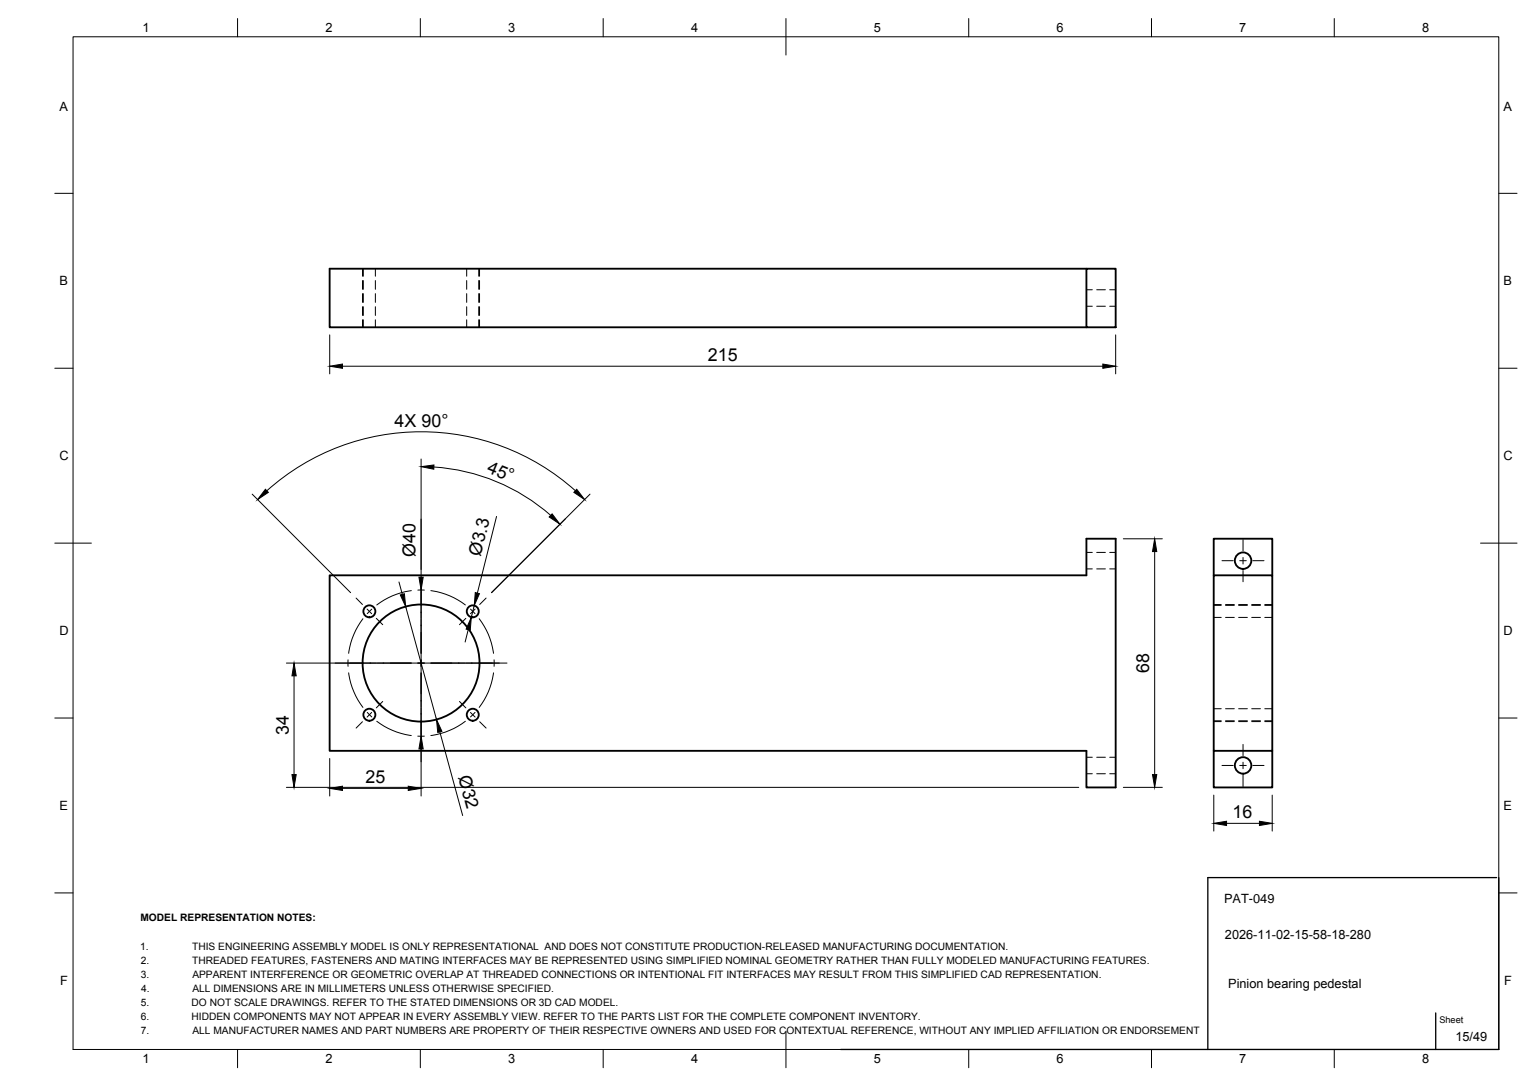
ISO-10303-21;
HEADER;
/* Generated by software containing ST-Developer
 * from STEP Tools, Inc. (www.steptools.com) 
 */

FILE_DESCRIPTION(
/* description */ ('Hand drill press frame (manual)'),
/* implementation_level */ '2;1');

FILE_NAME(
/* name */ 'Pinion bearing pedestal.step',
/* time_stamp */ '2026-10-28T03:25:28-07:00',
/* author */ (''),
/* organization */ (''),
/* preprocessor_version */ 'ST-DEVELOPER v20.2',
/* originating_system */ 'Autodesk Translation Framework v15.17.0.0',
/* authorisation */ '');

FILE_SCHEMA (('AUTOMOTIVE_DESIGN { 1 0 10303 214 3 1 1 }'));
ENDSEC;

DATA;
#10=MECHANICAL_DESIGN_GEOMETRIC_PRESENTATION_REPRESENTATION('',(#629),#33299);
#539=SHAPE_REPRESENTATION_RELATIONSHIP('SRR','None',#33498,#584);
#584=ADVANCED_BREP_SHAPE_REPRESENTATION('',(#681),#33260);
#629=STYLED_ITEM('',(#33814),#681);
#681=MANIFOLD_SOLID_BREP('Body1',#12647);
#764=FACE_BOUND('',#2219,.T.);
#765=FACE_BOUND('',#2221,.T.);
#766=FACE_BOUND('',#2225,.T.);
#767=FACE_BOUND('',#2226,.T.);
#768=FACE_BOUND('',#2227,.T.);
#769=FACE_BOUND('',#2228,.T.);
#770=FACE_BOUND('',#2229,.T.);
#771=FACE_BOUND('',#2232,.T.);
#772=FACE_BOUND('',#2233,.T.);
#773=FACE_BOUND('',#2234,.T.);
#774=FACE_BOUND('',#2235,.T.);
#775=FACE_BOUND('',#2236,.T.);
#776=FACE_BOUND('',#2240,.T.);
#777=FACE_BOUND('',#2241,.T.);
#983=PLANE('',#13453);
#984=PLANE('',#13454);
#985=PLANE('',#13455);
#986=PLANE('',#13456);
#987=PLANE('',#13457);
#988=PLANE('',#13458);
#989=PLANE('',#13459);
#990=PLANE('',#13460);
#991=PLANE('',#13461);
#992=PLANE('',#13462);
#1478=FACE_OUTER_BOUND('',#2211,.T.);
#1479=FACE_OUTER_BOUND('',#2212,.T.);
#1480=FACE_OUTER_BOUND('',#2213,.T.);
#1481=FACE_OUTER_BOUND('',#2214,.T.);
#1482=FACE_OUTER_BOUND('',#2215,.T.);
#1483=FACE_OUTER_BOUND('',#2216,.T.);
#1484=FACE_OUTER_BOUND('',#2217,.T.);
#1485=FACE_OUTER_BOUND('',#2218,.T.);
#1486=FACE_OUTER_BOUND('',#2220,.T.);
#1487=FACE_OUTER_BOUND('',#2222,.T.);
#1488=FACE_OUTER_BOUND('',#2223,.T.);
#1489=FACE_OUTER_BOUND('',#2224,.T.);
#1490=FACE_OUTER_BOUND('',#2230,.T.);
#1491=FACE_OUTER_BOUND('',#2231,.T.);
#1492=FACE_OUTER_BOUND('',#2237,.T.);
#1493=FACE_OUTER_BOUND('',#2238,.T.);
#1494=FACE_OUTER_BOUND('',#2239,.T.);
#2211=EDGE_LOOP('',(#9089,#9090,#9091,#9092));
#2212=EDGE_LOOP('',(#9093,#9094,#9095,#9096));
#2213=EDGE_LOOP('',(#9097,#9098,#9099,#9100));
#2214=EDGE_LOOP('',(#9101,#9102,#9103,#9104));
#2215=EDGE_LOOP('',(#9105,#9106,#9107,#9108));
#2216=EDGE_LOOP('',(#9109,#9110,#9111,#9112));
#2217=EDGE_LOOP('',(#9113,#9114,#9115,#9116));
#2218=EDGE_LOOP('',(#9117,#9118,#9119,#9120));
#2219=EDGE_LOOP('',(#9121));
#2220=EDGE_LOOP('',(#9122,#9123,#9124,#9125));
#2221=EDGE_LOOP('',(#9126));
#2222=EDGE_LOOP('',(#9127,#9128,#9129,#9130));
#2223=EDGE_LOOP('',(#9131,#9132,#9133,#9134));
#2224=EDGE_LOOP('',(#9135,#9136,#9137,#9138,#9139,#9140,#9141,#9142));
#2225=EDGE_LOOP('',(#9143));
#2226=EDGE_LOOP('',(#9144));
#2227=EDGE_LOOP('',(#9145));
#2228=EDGE_LOOP('',(#9146));
#2229=EDGE_LOOP('',(#9147));
#2230=EDGE_LOOP('',(#9148,#9149,#9150,#9151));
#2231=EDGE_LOOP('',(#9152,#9153,#9154,#9155,#9156,#9157,#9158,#9159));
#2232=EDGE_LOOP('',(#9160));
#2233=EDGE_LOOP('',(#9161));
#2234=EDGE_LOOP('',(#9162));
#2235=EDGE_LOOP('',(#9163));
#2236=EDGE_LOOP('',(#9164));
#2237=EDGE_LOOP('',(#9165,#9166,#9167,#9168));
#2238=EDGE_LOOP('',(#9169,#9170,#9171,#9172));
#2239=EDGE_LOOP('',(#9173,#9174,#9175,#9176));
#2240=EDGE_LOOP('',(#9177));
#2241=EDGE_LOOP('',(#9178));
#3111=LINE('',#18786,#4276);
#3112=LINE('',#18792,#4277);
#3113=LINE('',#18798,#4278);
#3114=LINE('',#18804,#4279);
#3115=LINE('',#18810,#4280);
#3116=LINE('',#18816,#4281);
#3117=LINE('',#18822,#4282);
#3118=LINE('',#18827,#4283);
#3119=LINE('',#18829,#4284);
#3120=LINE('',#18831,#4285);
#3121=LINE('',#18832,#4286);
#3122=LINE('',#18836,#4287);
#3123=LINE('',#18838,#4288);
#3124=LINE('',#18840,#4289);
#3125=LINE('',#18841,#4290);
#3126=LINE('',#18844,#4291);
#3127=LINE('',#18846,#4292);
#3128=LINE('',#18847,#4293);
#3129=LINE('',#18850,#4294);
#3130=LINE('',#18852,#4295);
#3131=LINE('',#18853,#4296);
#3132=LINE('',#18856,#4297);
#3133=LINE('',#18858,#4298);
#3134=LINE('',#18859,#4299);
#3135=LINE('',#18860,#4300);
#3136=LINE('',#18863,#4301);
#3137=LINE('',#18864,#4302);
#3138=LINE('',#18867,#4303);
#3139=LINE('',#18868,#4304);
#3140=LINE('',#18869,#4305);
#3141=LINE('',#18871,#4306);
#4276=VECTOR('',#15086,0.165);
#4277=VECTOR('',#15093,0.165);
#4278=VECTOR('',#15100,0.165);
#4279=VECTOR('',#15107,0.165);
#4280=VECTOR('',#15114,0.225);
#4281=VECTOR('',#15121,0.225);
#4282=VECTOR('',#15128,1.6);
#4283=VECTOR('',#15133,1.);
#4284=VECTOR('',#15134,1.);
#4285=VECTOR('',#15135,1.);
#4286=VECTOR('',#15136,1.);
#4287=VECTOR('',#15139,1.);
#4288=VECTOR('',#15140,1.);
#4289=VECTOR('',#15141,1.);
#4290=VECTOR('',#15142,1.);
#4291=VECTOR('',#15145,1.);
#4292=VECTOR('',#15146,1.);
#4293=VECTOR('',#15147,1.);
#4294=VECTOR('',#15150,1.);
#4295=VECTOR('',#15151,1.);
#4296=VECTOR('',#15152,1.);
#4297=VECTOR('',#15155,1.);
#4298=VECTOR('',#15156,1.);
#4299=VECTOR('',#15157,1.);
#4300=VECTOR('',#15158,1.);
#4301=VECTOR('',#15161,1.);
#4302=VECTOR('',#15162,1.);
#4303=VECTOR('',#15165,1.);
#4304=VECTOR('',#15166,1.);
#4305=VECTOR('',#15167,1.);
#4306=VECTOR('',#15170,1.);
#5306=CIRCLE('',#13433,0.165);
#5307=CIRCLE('',#13434,0.165);
#5308=CIRCLE('',#13436,0.165);
#5309=CIRCLE('',#13437,0.165);
#5310=CIRCLE('',#13439,0.165);
#5311=CIRCLE('',#13440,0.165);
#5312=CIRCLE('',#13442,0.165);
#5313=CIRCLE('',#13443,0.165);
#5314=CIRCLE('',#13445,0.225);
#5315=CIRCLE('',#13446,0.225);
#5316=CIRCLE('',#13448,0.225);
#5317=CIRCLE('',#13449,0.225);
#5318=CIRCLE('',#13451,1.6);
#5319=CIRCLE('',#13452,1.6);
#5836=VERTEX_POINT('',#18783);
#5837=VERTEX_POINT('',#18785);
#5838=VERTEX_POINT('',#18789);
#5839=VERTEX_POINT('',#18791);
#5840=VERTEX_POINT('',#18795);
#5841=VERTEX_POINT('',#18797);
#5842=VERTEX_POINT('',#18801);
#5843=VERTEX_POINT('',#18803);
#5844=VERTEX_POINT('',#18807);
#5845=VERTEX_POINT('',#18809);
#5846=VERTEX_POINT('',#18813);
#5847=VERTEX_POINT('',#18815);
#5848=VERTEX_POINT('',#18819);
#5849=VERTEX_POINT('',#18821);
#5850=VERTEX_POINT('',#18825);
#5851=VERTEX_POINT('',#18826);
#5852=VERTEX_POINT('',#18828);
#5853=VERTEX_POINT('',#18830);
#5854=VERTEX_POINT('',#18834);
#5855=VERTEX_POINT('',#18835);
#5856=VERTEX_POINT('',#18837);
#5857=VERTEX_POINT('',#18839);
#5858=VERTEX_POINT('',#18843);
#5859=VERTEX_POINT('',#18845);
#5860=VERTEX_POINT('',#18849);
#5861=VERTEX_POINT('',#18851);
#5862=VERTEX_POINT('',#18855);
#5863=VERTEX_POINT('',#18857);
#5864=VERTEX_POINT('',#18862);
#5865=VERTEX_POINT('',#18866);
#7073=EDGE_CURVE('',#5836,#5836,#5306,.T.);
#7074=EDGE_CURVE('',#5836,#5837,#3111,.T.);
#7075=EDGE_CURVE('',#5837,#5837,#5307,.T.);
#7076=EDGE_CURVE('',#5838,#5838,#5308,.T.);
#7077=EDGE_CURVE('',#5838,#5839,#3112,.T.);
#7078=EDGE_CURVE('',#5839,#5839,#5309,.T.);
#7079=EDGE_CURVE('',#5840,#5840,#5310,.T.);
#7080=EDGE_CURVE('',#5840,#5841,#3113,.T.);
#7081=EDGE_CURVE('',#5841,#5841,#5311,.T.);
#7082=EDGE_CURVE('',#5842,#5842,#5312,.T.);
#7083=EDGE_CURVE('',#5842,#5843,#3114,.T.);
#7084=EDGE_CURVE('',#5843,#5843,#5313,.T.);
#7085=EDGE_CURVE('',#5844,#5844,#5314,.T.);
#7086=EDGE_CURVE('',#5844,#5845,#3115,.T.);
#7087=EDGE_CURVE('',#5845,#5845,#5315,.T.);
#7088=EDGE_CURVE('',#5846,#5846,#5316,.T.);
#7089=EDGE_CURVE('',#5846,#5847,#3116,.T.);
#7090=EDGE_CURVE('',#5847,#5847,#5317,.T.);
#7091=EDGE_CURVE('',#5848,#5848,#5318,.T.);
#7092=EDGE_CURVE('',#5848,#5849,#3117,.T.);
#7093=EDGE_CURVE('',#5849,#5849,#5319,.T.);
#7094=EDGE_CURVE('',#5850,#5851,#3118,.T.);
#7095=EDGE_CURVE('',#5852,#5850,#3119,.T.);
#7096=EDGE_CURVE('',#5852,#5853,#3120,.T.);
#7097=EDGE_CURVE('',#5851,#5853,#3121,.T.);
#7098=EDGE_CURVE('',#5854,#5855,#3122,.T.);
#7099=EDGE_CURVE('',#5856,#5854,#3123,.T.);
#7100=EDGE_CURVE('',#5857,#5856,#3124,.T.);
#7101=EDGE_CURVE('',#5855,#5857,#3125,.T.);
#7102=EDGE_CURVE('',#5857,#5858,#3126,.T.);
#7103=EDGE_CURVE('',#5859,#5856,#3127,.T.);
#7104=EDGE_CURVE('',#5858,#5859,#3128,.T.);
#7105=EDGE_CURVE('',#5860,#5852,#3129,.T.);
#7106=EDGE_CURVE('',#5860,#5861,#3130,.T.);
#7107=EDGE_CURVE('',#5853,#5861,#3131,.T.);
#7108=EDGE_CURVE('',#5850,#5862,#3132,.T.);
#7109=EDGE_CURVE('',#5863,#5862,#3133,.T.);
#7110=EDGE_CURVE('',#5855,#5863,#3134,.T.);
#7111=EDGE_CURVE('',#5858,#5860,#3135,.T.);
#7112=EDGE_CURVE('',#5851,#5864,#3136,.T.);
#7113=EDGE_CURVE('',#5862,#5864,#3137,.T.);
#7114=EDGE_CURVE('',#5854,#5865,#3138,.T.);
#7115=EDGE_CURVE('',#5864,#5865,#3139,.T.);
#7116=EDGE_CURVE('',#5861,#5859,#3140,.T.);
#7117=EDGE_CURVE('',#5865,#5863,#3141,.T.);
#9089=ORIENTED_EDGE('',*,*,#7073,.F.);
#9090=ORIENTED_EDGE('',*,*,#7074,.T.);
#9091=ORIENTED_EDGE('',*,*,#7075,.F.);
#9092=ORIENTED_EDGE('',*,*,#7074,.F.);
#9093=ORIENTED_EDGE('',*,*,#7076,.F.);
#9094=ORIENTED_EDGE('',*,*,#7077,.T.);
#9095=ORIENTED_EDGE('',*,*,#7078,.F.);
#9096=ORIENTED_EDGE('',*,*,#7077,.F.);
#9097=ORIENTED_EDGE('',*,*,#7079,.F.);
#9098=ORIENTED_EDGE('',*,*,#7080,.T.);
#9099=ORIENTED_EDGE('',*,*,#7081,.F.);
#9100=ORIENTED_EDGE('',*,*,#7080,.F.);
#9101=ORIENTED_EDGE('',*,*,#7082,.F.);
#9102=ORIENTED_EDGE('',*,*,#7083,.T.);
#9103=ORIENTED_EDGE('',*,*,#7084,.F.);
#9104=ORIENTED_EDGE('',*,*,#7083,.F.);
#9105=ORIENTED_EDGE('',*,*,#7085,.F.);
#9106=ORIENTED_EDGE('',*,*,#7086,.T.);
#9107=ORIENTED_EDGE('',*,*,#7087,.F.);
#9108=ORIENTED_EDGE('',*,*,#7086,.F.);
#9109=ORIENTED_EDGE('',*,*,#7088,.F.);
#9110=ORIENTED_EDGE('',*,*,#7089,.T.);
#9111=ORIENTED_EDGE('',*,*,#7090,.F.);
#9112=ORIENTED_EDGE('',*,*,#7089,.F.);
#9113=ORIENTED_EDGE('',*,*,#7091,.F.);
#9114=ORIENTED_EDGE('',*,*,#7092,.T.);
#9115=ORIENTED_EDGE('',*,*,#7093,.F.);
#9116=ORIENTED_EDGE('',*,*,#7092,.F.);
#9117=ORIENTED_EDGE('',*,*,#7094,.F.);
#9118=ORIENTED_EDGE('',*,*,#7095,.F.);
#9119=ORIENTED_EDGE('',*,*,#7096,.T.);
#9120=ORIENTED_EDGE('',*,*,#7097,.F.);
#9121=ORIENTED_EDGE('',*,*,#7090,.T.);
#9122=ORIENTED_EDGE('',*,*,#7098,.F.);
#9123=ORIENTED_EDGE('',*,*,#7099,.F.);
#9124=ORIENTED_EDGE('',*,*,#7100,.F.);
#9125=ORIENTED_EDGE('',*,*,#7101,.F.);
#9126=ORIENTED_EDGE('',*,*,#7087,.T.);
#9127=ORIENTED_EDGE('',*,*,#7102,.F.);
#9128=ORIENTED_EDGE('',*,*,#7100,.T.);
#9129=ORIENTED_EDGE('',*,*,#7103,.F.);
#9130=ORIENTED_EDGE('',*,*,#7104,.F.);
#9131=ORIENTED_EDGE('',*,*,#7105,.F.);
#9132=ORIENTED_EDGE('',*,*,#7106,.T.);
#9133=ORIENTED_EDGE('',*,*,#7107,.F.);
#9134=ORIENTED_EDGE('',*,*,#7096,.F.);
#9135=ORIENTED_EDGE('',*,*,#7108,.T.);
#9136=ORIENTED_EDGE('',*,*,#7109,.F.);
#9137=ORIENTED_EDGE('',*,*,#7110,.F.);
#9138=ORIENTED_EDGE('',*,*,#7101,.T.);
#9139=ORIENTED_EDGE('',*,*,#7102,.T.);
#9140=ORIENTED_EDGE('',*,*,#7111,.T.);
#9141=ORIENTED_EDGE('',*,*,#7105,.T.);
#9142=ORIENTED_EDGE('',*,*,#7095,.T.);
#9143=ORIENTED_EDGE('',*,*,#7091,.T.);
#9144=ORIENTED_EDGE('',*,*,#7082,.T.);
#9145=ORIENTED_EDGE('',*,*,#7079,.T.);
#9146=ORIENTED_EDGE('',*,*,#7076,.T.);
#9147=ORIENTED_EDGE('',*,*,#7073,.T.);
#9148=ORIENTED_EDGE('',*,*,#7094,.T.);
#9149=ORIENTED_EDGE('',*,*,#7112,.T.);
#9150=ORIENTED_EDGE('',*,*,#7113,.F.);
#9151=ORIENTED_EDGE('',*,*,#7108,.F.);
#9152=ORIENTED_EDGE('',*,*,#7114,.T.);
#9153=ORIENTED_EDGE('',*,*,#7115,.F.);
#9154=ORIENTED_EDGE('',*,*,#7112,.F.);
#9155=ORIENTED_EDGE('',*,*,#7097,.T.);
#9156=ORIENTED_EDGE('',*,*,#7107,.T.);
#9157=ORIENTED_EDGE('',*,*,#7116,.T.);
#9158=ORIENTED_EDGE('',*,*,#7103,.T.);
#9159=ORIENTED_EDGE('',*,*,#7099,.T.);
#9160=ORIENTED_EDGE('',*,*,#7093,.T.);
#9161=ORIENTED_EDGE('',*,*,#7084,.T.);
#9162=ORIENTED_EDGE('',*,*,#7081,.T.);
#9163=ORIENTED_EDGE('',*,*,#7078,.T.);
#9164=ORIENTED_EDGE('',*,*,#7075,.T.);
#9165=ORIENTED_EDGE('',*,*,#7098,.T.);
#9166=ORIENTED_EDGE('',*,*,#7110,.T.);
#9167=ORIENTED_EDGE('',*,*,#7117,.F.);
#9168=ORIENTED_EDGE('',*,*,#7114,.F.);
#9169=ORIENTED_EDGE('',*,*,#7117,.T.);
#9170=ORIENTED_EDGE('',*,*,#7109,.T.);
#9171=ORIENTED_EDGE('',*,*,#7113,.T.);
#9172=ORIENTED_EDGE('',*,*,#7115,.T.);
#9173=ORIENTED_EDGE('',*,*,#7116,.F.);
#9174=ORIENTED_EDGE('',*,*,#7106,.F.);
#9175=ORIENTED_EDGE('',*,*,#7111,.F.);
#9176=ORIENTED_EDGE('',*,*,#7104,.T.);
#9177=ORIENTED_EDGE('',*,*,#7085,.T.);
#9178=ORIENTED_EDGE('',*,*,#7088,.T.);
#11828=CYLINDRICAL_SURFACE('',#13432,0.165);
#11829=CYLINDRICAL_SURFACE('',#13435,0.165);
#11830=CYLINDRICAL_SURFACE('',#13438,0.165);
#11831=CYLINDRICAL_SURFACE('',#13441,0.165);
#11832=CYLINDRICAL_SURFACE('',#13444,0.225);
#11833=CYLINDRICAL_SURFACE('',#13447,0.225);
#11834=CYLINDRICAL_SURFACE('',#13450,1.6);
#12087=ADVANCED_FACE('',(#1478),#11828,.F.);
#12088=ADVANCED_FACE('',(#1479),#11829,.F.);
#12089=ADVANCED_FACE('',(#1480),#11830,.F.);
#12090=ADVANCED_FACE('',(#1481),#11831,.F.);
#12091=ADVANCED_FACE('',(#1482),#11832,.F.);
#12092=ADVANCED_FACE('',(#1483),#11833,.F.);
#12093=ADVANCED_FACE('',(#1484),#11834,.F.);
#12094=ADVANCED_FACE('',(#1485,#764),#983,.T.);
#12095=ADVANCED_FACE('',(#1486,#765),#984,.T.);
#12096=ADVANCED_FACE('',(#1487),#985,.T.);
#12097=ADVANCED_FACE('',(#1488),#986,.T.);
#12098=ADVANCED_FACE('',(#1489,#766,#767,#768,#769,#770),#987,.T.);
#12099=ADVANCED_FACE('',(#1490),#988,.T.);
#12100=ADVANCED_FACE('',(#1491,#771,#772,#773,#774,#775),#989,.T.);
#12101=ADVANCED_FACE('',(#1492),#990,.T.);
#12102=ADVANCED_FACE('',(#1493),#991,.T.);
#12103=ADVANCED_FACE('',(#1494,#776,#777),#992,.F.);
#12647=CLOSED_SHELL('',(#12087,#12088,#12089,#12090,#12091,#12092,#12093,
#12094,#12095,#12096,#12097,#12098,#12099,#12100,#12101,#12102,#12103));
#13431=AXIS2_PLACEMENT_3D('',#18781,#15080,#15081);
#13432=AXIS2_PLACEMENT_3D('',#18782,#15082,#15083);
#13433=AXIS2_PLACEMENT_3D('',#18784,#15084,#15085);
#13434=AXIS2_PLACEMENT_3D('',#18787,#15087,#15088);
#13435=AXIS2_PLACEMENT_3D('',#18788,#15089,#15090);
#13436=AXIS2_PLACEMENT_3D('',#18790,#15091,#15092);
#13437=AXIS2_PLACEMENT_3D('',#18793,#15094,#15095);
#13438=AXIS2_PLACEMENT_3D('',#18794,#15096,#15097);
#13439=AXIS2_PLACEMENT_3D('',#18796,#15098,#15099);
#13440=AXIS2_PLACEMENT_3D('',#18799,#15101,#15102);
#13441=AXIS2_PLACEMENT_3D('',#18800,#15103,#15104);
#13442=AXIS2_PLACEMENT_3D('',#18802,#15105,#15106);
#13443=AXIS2_PLACEMENT_3D('',#18805,#15108,#15109);
#13444=AXIS2_PLACEMENT_3D('',#18806,#15110,#15111);
#13445=AXIS2_PLACEMENT_3D('',#18808,#15112,#15113);
#13446=AXIS2_PLACEMENT_3D('',#18811,#15115,#15116);
#13447=AXIS2_PLACEMENT_3D('',#18812,#15117,#15118);
#13448=AXIS2_PLACEMENT_3D('',#18814,#15119,#15120);
#13449=AXIS2_PLACEMENT_3D('',#18817,#15122,#15123);
#13450=AXIS2_PLACEMENT_3D('',#18818,#15124,#15125);
#13451=AXIS2_PLACEMENT_3D('',#18820,#15126,#15127);
#13452=AXIS2_PLACEMENT_3D('',#18823,#15129,#15130);
#13453=AXIS2_PLACEMENT_3D('',#18824,#15131,#15132);
#13454=AXIS2_PLACEMENT_3D('',#18833,#15137,#15138);
#13455=AXIS2_PLACEMENT_3D('',#18842,#15143,#15144);
#13456=AXIS2_PLACEMENT_3D('',#18848,#15148,#15149);
#13457=AXIS2_PLACEMENT_3D('',#18854,#15153,#15154);
#13458=AXIS2_PLACEMENT_3D('',#18861,#15159,#15160);
#13459=AXIS2_PLACEMENT_3D('',#18865,#15163,#15164);
#13460=AXIS2_PLACEMENT_3D('',#18870,#15168,#15169);
#13461=AXIS2_PLACEMENT_3D('',#18872,#15171,#15172);
#13462=AXIS2_PLACEMENT_3D('',#18873,#15173,#15174);
#15080=DIRECTION('axis',(0.,0.,1.));
#15081=DIRECTION('refdir',(1.,0.,0.));
#15082=DIRECTION('center_axis',(0.,1.,0.));
#15083=DIRECTION('ref_axis',(1.,0.,0.));
#15084=DIRECTION('center_axis',(0.,1.,0.));
#15085=DIRECTION('ref_axis',(1.,0.,0.));
#15086=DIRECTION('',(0.,1.,0.));
#15087=DIRECTION('center_axis',(0.,-1.,0.));
#15088=DIRECTION('ref_axis',(1.,0.,0.));
#15089=DIRECTION('center_axis',(0.,1.,0.));
#15090=DIRECTION('ref_axis',(1.,0.,0.));
#15091=DIRECTION('center_axis',(0.,1.,0.));
#15092=DIRECTION('ref_axis',(1.,0.,0.));
#15093=DIRECTION('',(0.,1.,0.));
#15094=DIRECTION('center_axis',(0.,-1.,0.));
#15095=DIRECTION('ref_axis',(1.,0.,0.));
#15096=DIRECTION('center_axis',(0.,1.,0.));
#15097=DIRECTION('ref_axis',(1.,0.,0.));
#15098=DIRECTION('center_axis',(0.,1.,0.));
#15099=DIRECTION('ref_axis',(1.,0.,0.));
#15100=DIRECTION('',(0.,1.,0.));
#15101=DIRECTION('center_axis',(0.,-1.,0.));
#15102=DIRECTION('ref_axis',(1.,0.,0.));
#15103=DIRECTION('center_axis',(0.,1.,0.));
#15104=DIRECTION('ref_axis',(1.,0.,0.));
#15105=DIRECTION('center_axis',(0.,1.,0.));
#15106=DIRECTION('ref_axis',(1.,0.,0.));
#15107=DIRECTION('',(0.,1.,0.));
#15108=DIRECTION('center_axis',(0.,-1.,0.));
#15109=DIRECTION('ref_axis',(1.,0.,0.));
#15110=DIRECTION('center_axis',(0.,0.,1.));
#15111=DIRECTION('ref_axis',(1.,0.,0.));
#15112=DIRECTION('center_axis',(0.,0.,1.));
#15113=DIRECTION('ref_axis',(1.,0.,0.));
#15114=DIRECTION('',(0.,0.,1.));
#15115=DIRECTION('center_axis',(0.,0.,-1.));
#15116=DIRECTION('ref_axis',(1.,0.,0.));
#15117=DIRECTION('center_axis',(0.,0.,1.));
#15118=DIRECTION('ref_axis',(1.,0.,0.));
#15119=DIRECTION('center_axis',(0.,0.,1.));
#15120=DIRECTION('ref_axis',(1.,0.,0.));
#15121=DIRECTION('',(0.,0.,1.));
#15122=DIRECTION('center_axis',(0.,0.,-1.));
#15123=DIRECTION('ref_axis',(1.,0.,0.));
#15124=DIRECTION('center_axis',(0.,1.,0.));
#15125=DIRECTION('ref_axis',(1.,0.,0.));
#15126=DIRECTION('center_axis',(0.,1.,0.));
#15127=DIRECTION('ref_axis',(1.,0.,0.));
#15128=DIRECTION('',(0.,1.,0.));
#15129=DIRECTION('center_axis',(0.,-1.,0.));
#15130=DIRECTION('ref_axis',(1.,0.,0.));
#15131=DIRECTION('center_axis',(0.,0.,1.));
#15132=DIRECTION('ref_axis',(1.,0.,0.));
#15133=DIRECTION('',(0.,1.,0.));
#15134=DIRECTION('',(-1.,0.,0.));
#15135=DIRECTION('',(0.,1.,0.));
#15136=DIRECTION('',(1.,0.,0.));
#15137=DIRECTION('center_axis',(0.,0.,1.));
#15138=DIRECTION('ref_axis',(1.,0.,0.));
#15139=DIRECTION('',(0.,-1.,0.));
#15140=DIRECTION('',(1.,0.,0.));
#15141=DIRECTION('',(0.,1.,0.));
#15142=DIRECTION('',(-1.,0.,0.));
#15143=DIRECTION('center_axis',(-1.,0.,0.));
#15144=DIRECTION('ref_axis',(0.,0.,1.));
#15145=DIRECTION('',(0.,0.,-1.));
#15146=DIRECTION('',(0.,0.,1.));
#15147=DIRECTION('',(0.,1.,0.));
#15148=DIRECTION('center_axis',(1.,0.,0.));
#15149=DIRECTION('ref_axis',(0.,0.,-1.));
#15150=DIRECTION('',(0.,0.,1.));
#15151=DIRECTION('',(0.,1.,0.));
#15152=DIRECTION('',(0.,0.,-1.));
#15153=DIRECTION('center_axis',(0.,-1.,0.));
#15154=DIRECTION('ref_axis',(1.,0.,0.));
#15155=DIRECTION('',(0.,0.,1.));
#15156=DIRECTION('',(1.,0.,0.));
#15157=DIRECTION('',(0.,0.,1.));
#15158=DIRECTION('',(1.,0.,0.));
#15159=DIRECTION('center_axis',(1.,0.,0.));
#15160=DIRECTION('ref_axis',(0.,1.,0.));
#15161=DIRECTION('',(0.,0.,1.));
#15162=DIRECTION('',(0.,1.,0.));
#15163=DIRECTION('center_axis',(0.,1.,0.));
#15164=DIRECTION('ref_axis',(-1.,0.,0.));
#15165=DIRECTION('',(0.,0.,1.));
#15166=DIRECTION('',(-1.,0.,0.));
#15167=DIRECTION('',(-1.,0.,0.));
#15168=DIRECTION('center_axis',(-1.,0.,0.));
#15169=DIRECTION('ref_axis',(0.,-1.,0.));
#15170=DIRECTION('',(0.,-1.,0.));
#15171=DIRECTION('center_axis',(0.,0.,1.));
#15172=DIRECTION('ref_axis',(1.,0.,0.));
#15173=DIRECTION('center_axis',(0.,0.,1.));
#15174=DIRECTION('ref_axis',(1.,0.,0.));
#18781=CARTESIAN_POINT('',(0.,0.,0.));
#18782=CARTESIAN_POINT('Origin',(-4.66421356237309,-3.9,18.5857864376269));
#18783=CARTESIAN_POINT('',(-4.82921356237309,-3.8,18.5857864376269));
#18784=CARTESIAN_POINT('Origin',(-4.66421356237309,-3.8,18.5857864376269));
#18785=CARTESIAN_POINT('',(-4.82921356237309,-2.2,18.5857864376269));
#18786=CARTESIAN_POINT('',(-4.82921356237309,-3.9,18.5857864376269));
#18787=CARTESIAN_POINT('Origin',(-4.66421356237309,-2.2,18.5857864376269));
#18788=CARTESIAN_POINT('Origin',(-4.66421356237309,-3.9,21.4142135623731));
#18789=CARTESIAN_POINT('',(-4.82921356237309,-3.8,21.4142135623731));
#18790=CARTESIAN_POINT('Origin',(-4.66421356237309,-3.8,21.4142135623731));
#18791=CARTESIAN_POINT('',(-4.82921356237309,-2.2,21.4142135623731));
#18792=CARTESIAN_POINT('',(-4.82921356237309,-3.9,21.4142135623731));
#18793=CARTESIAN_POINT('Origin',(-4.66421356237309,-2.2,21.4142135623731));
#18794=CARTESIAN_POINT('Origin',(-1.8357864376269,-3.9,21.4142135623731));
#18795=CARTESIAN_POINT('',(-2.00078643762691,-3.8,21.4142135623731));
#18796=CARTESIAN_POINT('Origin',(-1.8357864376269,-3.8,21.4142135623731));
#18797=CARTESIAN_POINT('',(-2.00078643762691,-2.2,21.4142135623731));
#18798=CARTESIAN_POINT('',(-2.00078643762691,-3.9,21.4142135623731));
#18799=CARTESIAN_POINT('Origin',(-1.8357864376269,-2.2,21.4142135623731));
#18800=CARTESIAN_POINT('Origin',(-1.83578643762691,-3.9,18.5857864376269));
#18801=CARTESIAN_POINT('',(-2.00078643762691,-3.8,18.5857864376269));
#18802=CARTESIAN_POINT('Origin',(-1.83578643762691,-3.8,18.5857864376269));
#18803=CARTESIAN_POINT('',(-2.00078643762691,-2.2,18.5857864376269));
#18804=CARTESIAN_POINT('',(-2.00078643762691,-3.9,18.5857864376269));
#18805=CARTESIAN_POINT('Origin',(-1.83578643762691,-2.2,18.5857864376269));
#18806=CARTESIAN_POINT('Origin',(-6.05,-3.,0.9));
#18807=CARTESIAN_POINT('',(-6.275,-3.,1.));
#18808=CARTESIAN_POINT('Origin',(-6.05,-3.,1.));
#18809=CARTESIAN_POINT('',(-6.275,-3.,1.8));
#18810=CARTESIAN_POINT('',(-6.275,-3.,0.9));
#18811=CARTESIAN_POINT('Origin',(-6.05,-3.,1.8));
#18812=CARTESIAN_POINT('Origin',(-0.45,-3.,0.9));
#18813=CARTESIAN_POINT('',(-0.675,-3.,1.));
#18814=CARTESIAN_POINT('Origin',(-0.45,-3.,1.));
#18815=CARTESIAN_POINT('',(-0.675,-3.,1.8));
#18816=CARTESIAN_POINT('',(-0.675,-3.,0.9));
#18817=CARTESIAN_POINT('Origin',(-0.45,-3.,1.8));
#18818=CARTESIAN_POINT('Origin',(-3.25,-3.9,20.));
#18819=CARTESIAN_POINT('',(-4.85,-3.8,20.));
#18820=CARTESIAN_POINT('Origin',(-3.25,-3.8,20.));
#18821=CARTESIAN_POINT('',(-4.85,-2.2,20.));
#18822=CARTESIAN_POINT('',(-4.85,-3.9,20.));
#18823=CARTESIAN_POINT('Origin',(-3.25,-2.2,20.));
#18824=CARTESIAN_POINT('Origin',(-6.65,-3.8,1.8));
#18825=CARTESIAN_POINT('',(-0.85,-3.8,1.8));
#18826=CARTESIAN_POINT('',(-0.85,-2.2,1.8));
#18827=CARTESIAN_POINT('',(-0.85,-3.8,1.8));
#18828=CARTESIAN_POINT('',(0.15,-3.8,1.8));
#18829=CARTESIAN_POINT('',(0.15,-3.8,1.8));
#18830=CARTESIAN_POINT('',(0.15,-2.2,1.8));
#18831=CARTESIAN_POINT('',(0.15,-3.8,1.8));
#18832=CARTESIAN_POINT('',(0.15,-2.2,1.8));
#18833=CARTESIAN_POINT('Origin',(-6.65,-3.8,1.8));
#18834=CARTESIAN_POINT('',(-5.65,-2.2,1.8));
#18835=CARTESIAN_POINT('',(-5.65,-3.8,1.8));
#18836=CARTESIAN_POINT('',(-5.65,-3.,1.8));
#18837=CARTESIAN_POINT('',(-6.65,-2.2,1.8));
#18838=CARTESIAN_POINT('',(0.15,-2.2,1.8));
#18839=CARTESIAN_POINT('',(-6.65,-3.8,1.8));
#18840=CARTESIAN_POINT('',(-6.65,-3.8,1.8));
#18841=CARTESIAN_POINT('',(0.15,-3.8,1.8));
#18842=CARTESIAN_POINT('Origin',(-6.65,-3.8,1.));
#18843=CARTESIAN_POINT('',(-6.65,-3.8,1.));
#18844=CARTESIAN_POINT('',(-6.65,-3.8,1.8));
#18845=CARTESIAN_POINT('',(-6.65,-2.2,1.));
#18846=CARTESIAN_POINT('',(-6.65,-2.2,1.8));
#18847=CARTESIAN_POINT('',(-6.65,-3.8,1.));
#18848=CARTESIAN_POINT('Origin',(0.15,-3.8,1.8));
#18849=CARTESIAN_POINT('',(0.15,-3.8,1.));
#18850=CARTESIAN_POINT('',(0.15,-3.8,1.));
#18851=CARTESIAN_POINT('',(0.15,-2.2,1.));
#18852=CARTESIAN_POINT('',(0.15,-3.8,1.));
#18853=CARTESIAN_POINT('',(0.15,-2.2,1.));
#18854=CARTESIAN_POINT('Origin',(-5.65,-3.8,1.));
#18855=CARTESIAN_POINT('',(-0.85,-3.8,22.5));
#18856=CARTESIAN_POINT('',(-0.85,-3.8,1.));
#18857=CARTESIAN_POINT('',(-5.65,-3.8,22.5));
#18858=CARTESIAN_POINT('',(-5.65,-3.8,22.5));
#18859=CARTESIAN_POINT('',(-5.65,-3.8,1.));
#18860=CARTESIAN_POINT('',(-6.65,-3.8,1.));
#18861=CARTESIAN_POINT('Origin',(-0.85,-3.8,1.));
#18862=CARTESIAN_POINT('',(-0.85,-2.2,22.5));
#18863=CARTESIAN_POINT('',(-0.85,-2.2,1.));
#18864=CARTESIAN_POINT('',(-0.85,-3.8,22.5));
#18865=CARTESIAN_POINT('Origin',(-0.85,-2.2,1.));
#18866=CARTESIAN_POINT('',(-5.65,-2.2,22.5));
#18867=CARTESIAN_POINT('',(-5.65,-2.2,1.));
#18868=CARTESIAN_POINT('',(-0.85,-2.2,22.5));
#18869=CARTESIAN_POINT('',(-6.65,-2.2,1.));
#18870=CARTESIAN_POINT('Origin',(-5.65,-2.2,1.));
#18871=CARTESIAN_POINT('',(-5.65,-2.2,22.5));
#18872=CARTESIAN_POINT('Origin',(-3.25,-3.,22.5));
#18873=CARTESIAN_POINT('Origin',(-3.25,-3.,1.));
#33208=UNCERTAINTY_MEASURE_WITH_UNIT(LENGTH_MEASURE(0.001),#33300,
'DISTANCE_ACCURACY_VALUE',
'Maximum model space distance between geometric entities at asserted c
onnectivities');
#33247=UNCERTAINTY_MEASURE_WITH_UNIT(LENGTH_MEASURE(0.001),#33300,
'DISTANCE_ACCURACY_VALUE',
'Maximum model space distance between geometric entities at asserted c
onnectivities');
#33260=(
GEOMETRIC_REPRESENTATION_CONTEXT(3)
GLOBAL_UNCERTAINTY_ASSIGNED_CONTEXT((#33208))
GLOBAL_UNIT_ASSIGNED_CONTEXT((#33300,#33302,#33303))
REPRESENTATION_CONTEXT('','3D')
);
#33299=(
GEOMETRIC_REPRESENTATION_CONTEXT(3)
GLOBAL_UNCERTAINTY_ASSIGNED_CONTEXT((#33247))
GLOBAL_UNIT_ASSIGNED_CONTEXT((#33300,#33302,#33303))
REPRESENTATION_CONTEXT('','3D')
);
#33300=(
LENGTH_UNIT()
NAMED_UNIT(*)
SI_UNIT(.CENTI.,.METRE.)
);
#33302=(
NAMED_UNIT(*)
PLANE_ANGLE_UNIT()
SI_UNIT($,.RADIAN.)
);
#33303=(
NAMED_UNIT(*)
SI_UNIT($,.STERADIAN.)
SOLID_ANGLE_UNIT()
);
#33316=SHAPE_DEFINITION_REPRESENTATION(#33367,#33498);
#33367=PRODUCT_DEFINITION_SHAPE('',$,#33550);
#33498=SHAPE_REPRESENTATION('',(#13431),#33260);
#33537=PRODUCT_DEFINITION_CONTEXT('part definition',#33692,'design');
#33550=PRODUCT_DEFINITION('Pinion bearing pedestal',
'Pinion bearing pedestal',#33601,#33537);
#33601=PRODUCT_DEFINITION_FORMATION('',$,#33706);
#33692=APPLICATION_CONTEXT(
'Core Data for Automotive Mechanical Design Process');
#33693=PRODUCT_CONTEXT('part definition',#33692,'mechanical');
#33706=PRODUCT('Pinion bearing pedestal','Pinion bearing pedestal',
'Pinion bearing pedestal',(#33693));
#33808=COLOUR_RGB('Grey',0.48,0.52,0.57);
#33809=FILL_AREA_STYLE_COLOUR('',#33808);
#33810=FILL_AREA_STYLE('',(#33809));
#33811=SURFACE_STYLE_FILL_AREA(#33810);
#33812=SURFACE_SIDE_STYLE('',(#33811));
#33813=SURFACE_STYLE_USAGE(.BOTH.,#33812);
#33814=PRESENTATION_STYLE_ASSIGNMENT((#33813));
ENDSEC;
END-ISO-10303-21;
